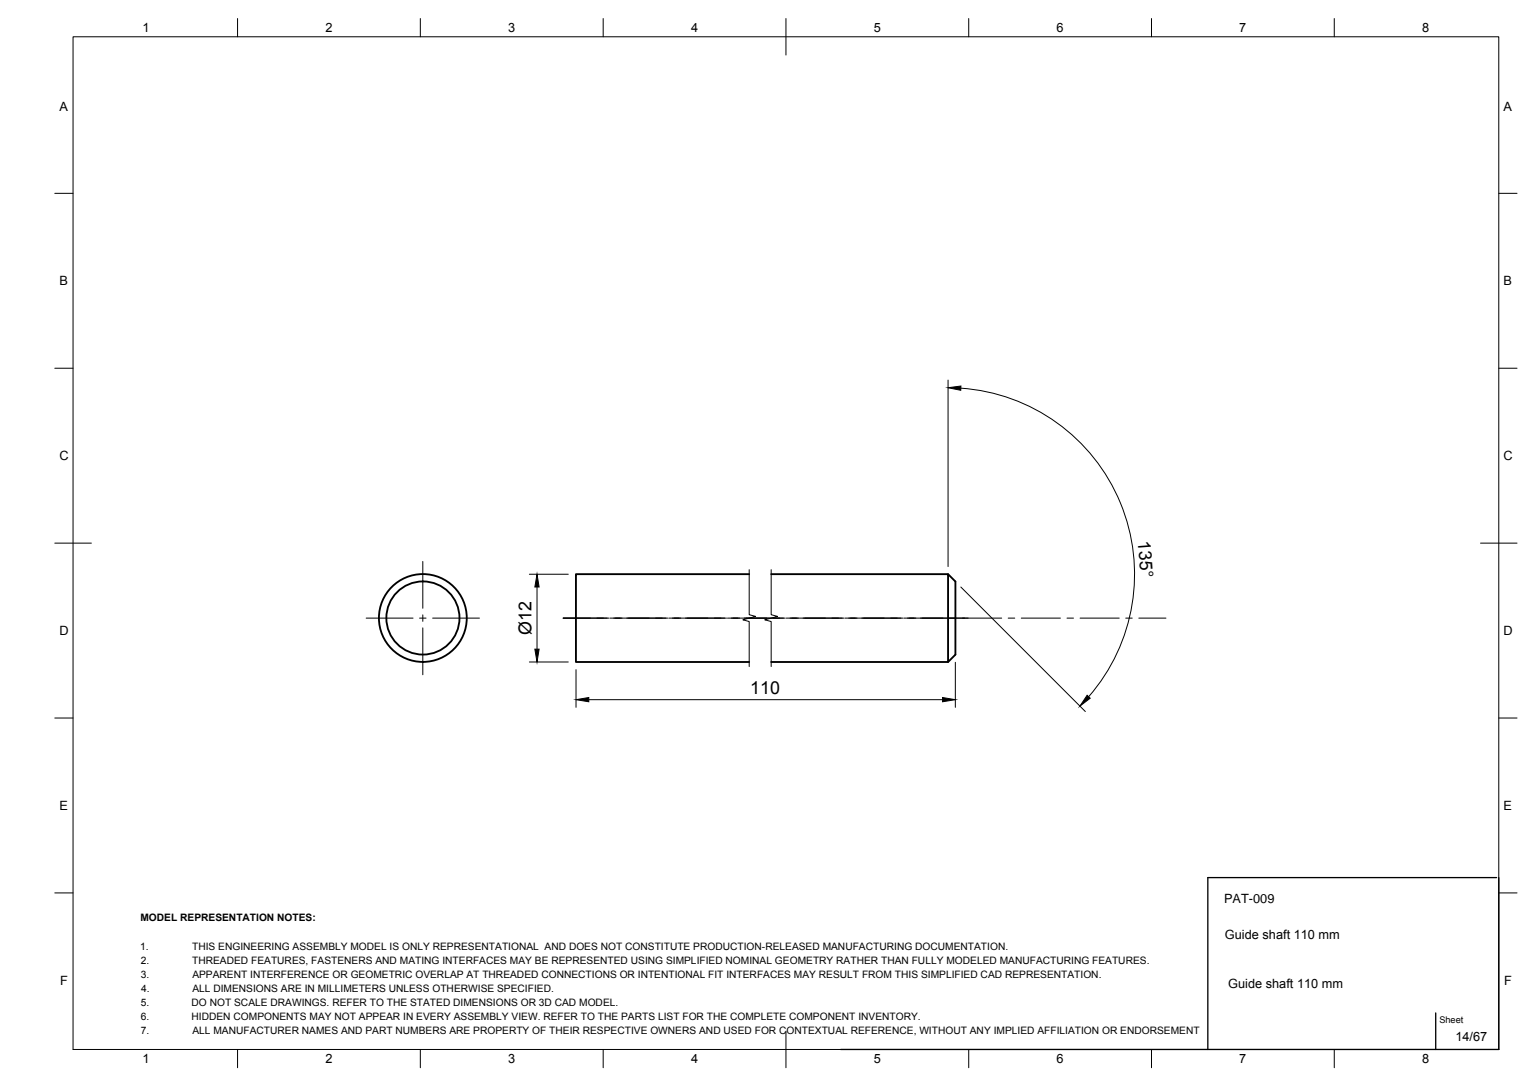
ISO-10303-21;
HEADER;
/* Generated by software containing ST-Developer
 * from STEP Tools, Inc. (www.steptools.com) 
 */

FILE_DESCRIPTION(
/* description */ ('Bell-crank linkage with push rods'),
/* implementation_level */ '2;1');

FILE_NAME(
/* name */ 'Guide shaft 110 mm.step',
/* time_stamp */ '2026-10-28T03:25:15-07:00',
/* author */ (''),
/* organization */ (''),
/* preprocessor_version */ 'ST-DEVELOPER v20.2',
/* originating_system */ 'Autodesk Translation Framework v15.17.0.0',
/* authorisation */ '');

FILE_SCHEMA (('AUTOMOTIVE_DESIGN { 1 0 10303 214 3 1 1 }'));
ENDSEC;

DATA;
#10=MECHANICAL_DESIGN_GEOMETRIC_PRESENTATION_REPRESENTATION('',(#627),#16678);
#440=CONICAL_SURFACE('',#9925,0.55,0.785398163397448);
#511=SHAPE_REPRESENTATION_RELATIONSHIP('SRR','None',#16928,#565);
#565=ADVANCED_BREP_SHAPE_REPRESENTATION('',(#688),#16633);
#627=STYLED_ITEM('',(#17291),#688);
#688=MANIFOLD_SOLID_BREP('Body1',#8818);
#1071=PLANE('',#9923);
#1072=PLANE('',#9929);
#1461=FACE_OUTER_BOUND('',#2080,.T.);
#1462=FACE_OUTER_BOUND('',#2081,.T.);
#1463=FACE_OUTER_BOUND('',#2082,.T.);
#1464=FACE_OUTER_BOUND('',#2083,.T.);
#2080=EDGE_LOOP('',(#6887));
#2081=EDGE_LOOP('',(#6888,#6889,#6890,#6891));
#2082=EDGE_LOOP('',(#6892,#6893,#6894,#6895));
#2083=EDGE_LOOP('',(#6896));
#2755=LINE('',#15069,#3304);
#2756=LINE('',#15072,#3305);
#3304=VECTOR('',#11799,0.55);
#3305=VECTOR('',#11804,0.6);
#3861=CIRCLE('',#9924,0.6);
#3862=CIRCLE('',#9926,0.6);
#3863=CIRCLE('',#9927,0.5);
#4443=VERTEX_POINT('',#15063);
#4444=VERTEX_POINT('',#15066);
#4445=VERTEX_POINT('',#15068);
#5321=EDGE_CURVE('',#4443,#4443,#3861,.T.);
#5322=EDGE_CURVE('',#4444,#4444,#3862,.T.);
#5323=EDGE_CURVE('',#4444,#4445,#2755,.T.);
#5324=EDGE_CURVE('',#4445,#4445,#3863,.T.);
#5325=EDGE_CURVE('',#4443,#4444,#2756,.T.);
#6887=ORIENTED_EDGE('',*,*,#5321,.F.);
#6888=ORIENTED_EDGE('',*,*,#5322,.T.);
#6889=ORIENTED_EDGE('',*,*,#5323,.T.);
#6890=ORIENTED_EDGE('',*,*,#5324,.T.);
#6891=ORIENTED_EDGE('',*,*,#5323,.F.);
#6892=ORIENTED_EDGE('',*,*,#5321,.T.);
#6893=ORIENTED_EDGE('',*,*,#5325,.T.);
#6894=ORIENTED_EDGE('',*,*,#5322,.F.);
#6895=ORIENTED_EDGE('',*,*,#5325,.F.);
#6896=ORIENTED_EDGE('',*,*,#5324,.F.);
#8151=CYLINDRICAL_SURFACE('',#9928,0.6);
#8486=ADVANCED_FACE('',(#1461),#1071,.T.);
#8487=ADVANCED_FACE('',(#1462),#440,.T.);
#8488=ADVANCED_FACE('',(#1463),#8151,.T.);
#8489=ADVANCED_FACE('',(#1464),#1072,.F.);
#8818=CLOSED_SHELL('',(#8486,#8487,#8488,#8489));
#9922=AXIS2_PLACEMENT_3D('',#15061,#11789,#11790);
#9923=AXIS2_PLACEMENT_3D('',#15062,#11791,#11792);
#9924=AXIS2_PLACEMENT_3D('',#15064,#11793,#11794);
#9925=AXIS2_PLACEMENT_3D('',#15065,#11795,#11796);
#9926=AXIS2_PLACEMENT_3D('',#15067,#11797,#11798);
#9927=AXIS2_PLACEMENT_3D('',#15070,#11800,#11801);
#9928=AXIS2_PLACEMENT_3D('',#15071,#11802,#11803);
#9929=AXIS2_PLACEMENT_3D('',#15073,#11805,#11806);
#11789=DIRECTION('axis',(0.,0.,1.));
#11790=DIRECTION('refdir',(1.,0.,0.));
#11791=DIRECTION('center_axis',(1.,0.,0.));
#11792=DIRECTION('ref_axis',(0.,0.,-1.));
#11793=DIRECTION('center_axis',(-1.,0.,0.));
#11794=DIRECTION('ref_axis',(0.,0.,-1.));
#11795=DIRECTION('center_axis',(1.,0.,0.));
#11796=DIRECTION('ref_axis',(0.,0.,-1.));
#11797=DIRECTION('center_axis',(-1.,0.,0.));
#11798=DIRECTION('ref_axis',(0.,0.,-1.));
#11799=DIRECTION('',(-0.707106781186548,8.65956056235493E-17,-0.707106781186547));
#11800=DIRECTION('center_axis',(1.,0.,0.));
#11801=DIRECTION('ref_axis',(0.,0.,-1.));
#11802=DIRECTION('center_axis',(1.,0.,0.));
#11803=DIRECTION('ref_axis',(0.,0.,-1.));
#11804=DIRECTION('',(-1.,0.,0.));
#11805=DIRECTION('center_axis',(1.,0.,0.));
#11806=DIRECTION('ref_axis',(0.,0.,-1.));
#15061=CARTESIAN_POINT('',(0.,0.,0.));
#15062=CARTESIAN_POINT('Origin',(11.,0.,0.));
#15063=CARTESIAN_POINT('',(11.,7.34788079488412E-17,0.6));
#15064=CARTESIAN_POINT('Origin',(11.,0.,0.));
#15065=CARTESIAN_POINT('Origin',(0.05,0.,0.));
#15066=CARTESIAN_POINT('',(0.1,7.34788079488412E-17,0.6));
#15067=CARTESIAN_POINT('Origin',(0.1,0.,0.));
#15068=CARTESIAN_POINT('',(0.,-6.12323399573677E-17,0.5));
#15069=CARTESIAN_POINT('',(0.05,-6.73555739531044E-17,0.55));
#15070=CARTESIAN_POINT('Origin',(0.,0.,0.));
#15071=CARTESIAN_POINT('Origin',(0.,0.,0.));
#15072=CARTESIAN_POINT('',(0.,-7.34788079488412E-17,0.6));
#15073=CARTESIAN_POINT('Origin',(0.,0.,0.));
#16569=UNCERTAINTY_MEASURE_WITH_UNIT(LENGTH_MEASURE(0.001),#16679,
'DISTANCE_ACCURACY_VALUE',
'Maximum model space distance between geometric entities at asserted c
onnectivities');
#16614=UNCERTAINTY_MEASURE_WITH_UNIT(LENGTH_MEASURE(0.001),#16679,
'DISTANCE_ACCURACY_VALUE',
'Maximum model space distance between geometric entities at asserted c
onnectivities');
#16633=(
GEOMETRIC_REPRESENTATION_CONTEXT(3)
GLOBAL_UNCERTAINTY_ASSIGNED_CONTEXT((#16569))
GLOBAL_UNIT_ASSIGNED_CONTEXT((#16679,#16681,#16682))
REPRESENTATION_CONTEXT('','3D')
);
#16678=(
GEOMETRIC_REPRESENTATION_CONTEXT(3)
GLOBAL_UNCERTAINTY_ASSIGNED_CONTEXT((#16614))
GLOBAL_UNIT_ASSIGNED_CONTEXT((#16679,#16681,#16682))
REPRESENTATION_CONTEXT('','3D')
);
#16679=(
LENGTH_UNIT()
NAMED_UNIT(*)
SI_UNIT(.CENTI.,.METRE.)
);
#16681=(
NAMED_UNIT(*)
PLANE_ANGLE_UNIT()
SI_UNIT($,.RADIAN.)
);
#16682=(
NAMED_UNIT(*)
SI_UNIT($,.STERADIAN.)
SOLID_ANGLE_UNIT()
);
#16701=SHAPE_DEFINITION_REPRESENTATION(#16769,#16928);
#16769=PRODUCT_DEFINITION_SHAPE('',$,#16992);
#16928=SHAPE_REPRESENTATION('',(#9922),#16633);
#16973=PRODUCT_DEFINITION_CONTEXT('part definition',#17164,'design');
#16992=PRODUCT_DEFINITION('Guide shaft 110 mm','Guide shaft 110 mm',#17055,
#16973);
#17055=PRODUCT_DEFINITION_FORMATION('',$,#17184);
#17164=APPLICATION_CONTEXT(
'Core Data for Automotive Mechanical Design Process');
#17165=PRODUCT_CONTEXT('part definition',#17164,'mechanical');
#17184=PRODUCT('Guide shaft 110 mm','Guide shaft 110 mm',
'Guide shaft 110 mm',(#17165));
#17285=COLOUR_RGB('Grey',0.48,0.52,0.57);
#17286=FILL_AREA_STYLE_COLOUR('',#17285);
#17287=FILL_AREA_STYLE('',(#17286));
#17288=SURFACE_STYLE_FILL_AREA(#17287);
#17289=SURFACE_SIDE_STYLE('',(#17288));
#17290=SURFACE_STYLE_USAGE(.BOTH.,#17289);
#17291=PRESENTATION_STYLE_ASSIGNMENT((#17290));
ENDSEC;
END-ISO-10303-21;
